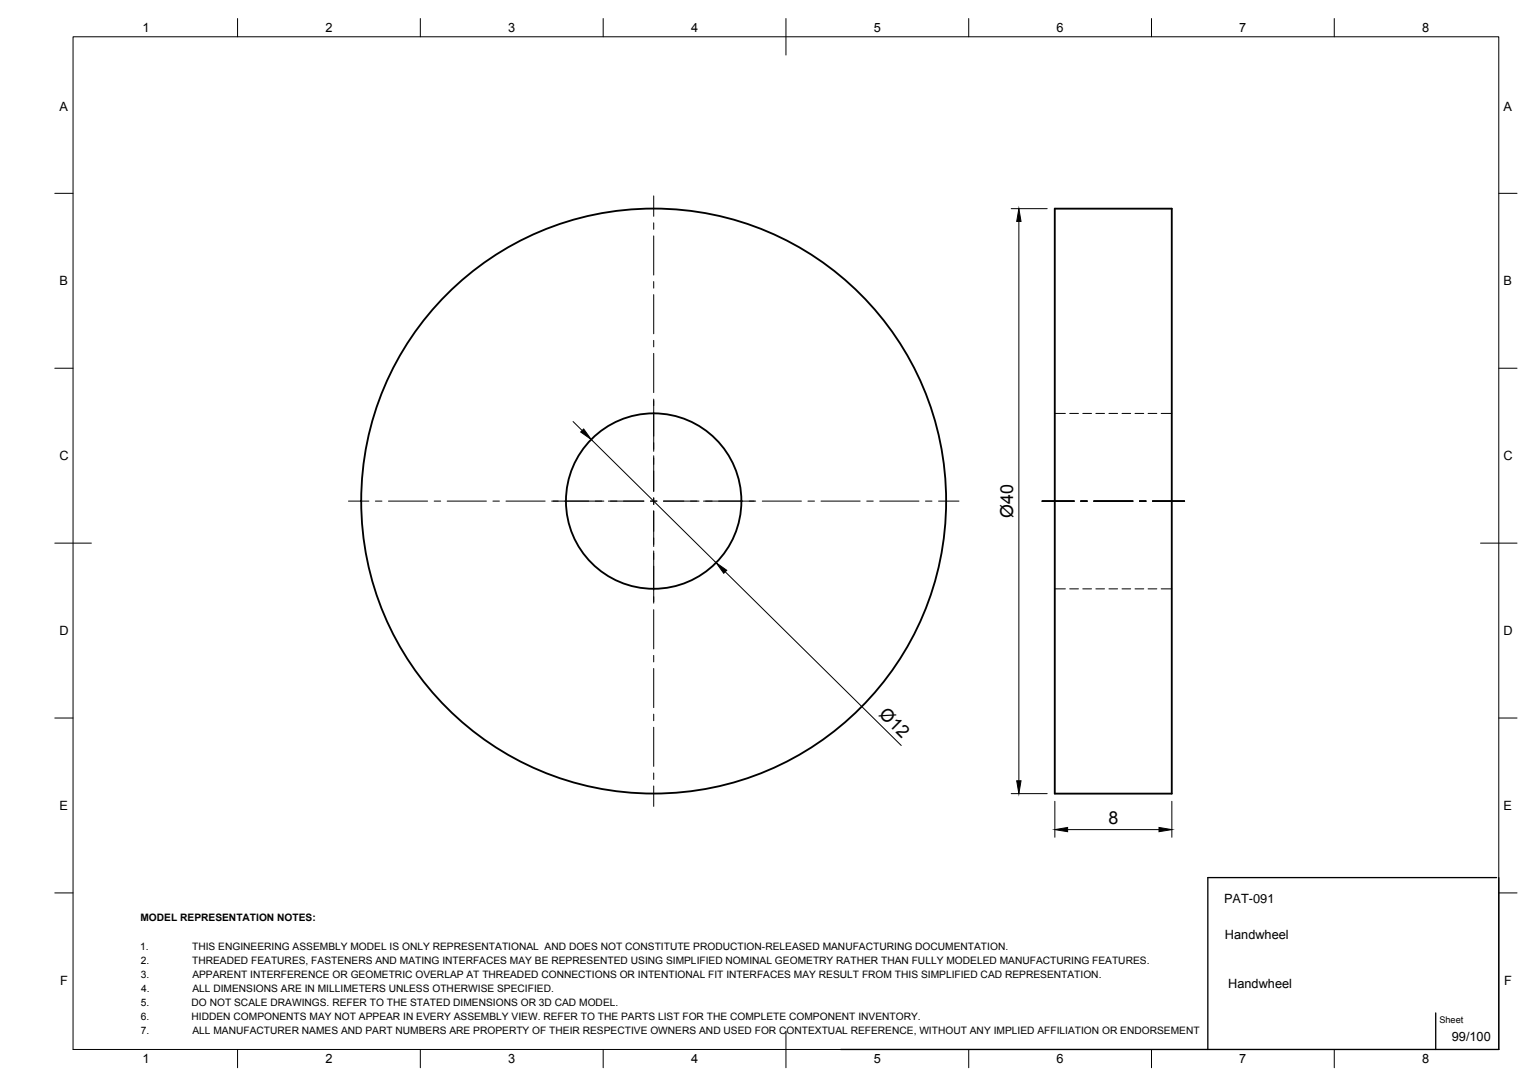
ISO-10303-21;
HEADER;
/* Generated by software containing ST-Developer
 * from STEP Tools, Inc. (www.steptools.com) 
 */

FILE_DESCRIPTION(
/* description */ ('PAT-091'),
/* implementation_level */ '2;1');

FILE_NAME(
/* name */ 'Handwheel.step',
/* time_stamp */ '2026-10-27T15:34:44-07:00',
/* author */ (''),
/* organization */ (''),
/* preprocessor_version */ 'ST-DEVELOPER v20.2',
/* originating_system */ 'Autodesk Translation Framework v15.17.0.0',
/* authorisation */ '');

FILE_SCHEMA (('AUTOMOTIVE_DESIGN { 1 0 10303 214 3 1 1 }'));
ENDSEC;

DATA;
#10=MECHANICAL_DESIGN_GEOMETRIC_PRESENTATION_REPRESENTATION('',(#1093),#25100);
#860=SHAPE_REPRESENTATION_RELATIONSHIP('SRR','None',#25629,#970);
#970=ADVANCED_BREP_SHAPE_REPRESENTATION('',(#1214),#25099);
#1093=STYLED_ITEM('',(#26184),#1214);
#1214=MANIFOLD_SOLID_BREP('Body1',#13373);
#1637=FACE_BOUND('',#4120,.T.);
#1638=FACE_BOUND('',#4122,.T.);
#1639=FACE_BOUND('',#4123,.T.);
#2060=PLANE('',#16445);
#2061=PLANE('',#16452);
#2062=PLANE('',#16453);
#2875=FACE_OUTER_BOUND('',#4115,.T.);
#2876=FACE_OUTER_BOUND('',#4116,.T.);
#2877=FACE_OUTER_BOUND('',#4117,.T.);
#2878=FACE_OUTER_BOUND('',#4118,.T.);
#2879=FACE_OUTER_BOUND('',#4119,.T.);
#2880=FACE_OUTER_BOUND('',#4121,.T.);
#4115=EDGE_LOOP('',(#12056,#12057,#12058,#12059));
#4116=EDGE_LOOP('',(#12060));
#4117=EDGE_LOOP('',(#12061,#12062,#12063,#12064));
#4118=EDGE_LOOP('',(#12065,#12066,#12067,#12068));
#4119=EDGE_LOOP('',(#12069));
#4120=EDGE_LOOP('',(#12070));
#4121=EDGE_LOOP('',(#12071));
#4122=EDGE_LOOP('',(#12072));
#4123=EDGE_LOOP('',(#12073));
#4861=LINE('',#24828,#5601);
#4862=LINE('',#24835,#5602);
#4863=LINE('',#24841,#5603);
#5601=VECTOR('',#20923,0.4);
#5602=VECTOR('',#20932,0.6);
#5603=VECTOR('',#20939,2.);
#6377=CIRCLE('',#16443,0.4);
#6378=CIRCLE('',#16444,0.4);
#6379=CIRCLE('',#16447,0.6);
#6380=CIRCLE('',#16448,0.6);
#6381=CIRCLE('',#16450,2.);
#6382=CIRCLE('',#16451,2.);
#7415=VERTEX_POINT('',#24825);
#7416=VERTEX_POINT('',#24827);
#7417=VERTEX_POINT('',#24832);
#7418=VERTEX_POINT('',#24834);
#7419=VERTEX_POINT('',#24838);
#7420=VERTEX_POINT('',#24840);
#8963=EDGE_CURVE('',#7415,#7415,#6377,.T.);
#8964=EDGE_CURVE('',#7415,#7416,#4861,.T.);
#8965=EDGE_CURVE('',#7416,#7416,#6378,.T.);
#8966=EDGE_CURVE('',#7417,#7417,#6379,.T.);
#8967=EDGE_CURVE('',#7417,#7418,#4862,.T.);
#8968=EDGE_CURVE('',#7418,#7418,#6380,.T.);
#8969=EDGE_CURVE('',#7419,#7419,#6381,.T.);
#8970=EDGE_CURVE('',#7419,#7420,#4863,.T.);
#8971=EDGE_CURVE('',#7420,#7420,#6382,.T.);
#12056=ORIENTED_EDGE('',*,*,#8963,.F.);
#12057=ORIENTED_EDGE('',*,*,#8964,.T.);
#12058=ORIENTED_EDGE('',*,*,#8965,.T.);
#12059=ORIENTED_EDGE('',*,*,#8964,.F.);
#12060=ORIENTED_EDGE('',*,*,#8965,.F.);
#12061=ORIENTED_EDGE('',*,*,#8966,.F.);
#12062=ORIENTED_EDGE('',*,*,#8967,.T.);
#12063=ORIENTED_EDGE('',*,*,#8968,.T.);
#12064=ORIENTED_EDGE('',*,*,#8967,.F.);
#12065=ORIENTED_EDGE('',*,*,#8969,.F.);
#12066=ORIENTED_EDGE('',*,*,#8970,.T.);
#12067=ORIENTED_EDGE('',*,*,#8971,.T.);
#12068=ORIENTED_EDGE('',*,*,#8970,.F.);
#12069=ORIENTED_EDGE('',*,*,#8969,.T.);
#12070=ORIENTED_EDGE('',*,*,#8966,.T.);
#12071=ORIENTED_EDGE('',*,*,#8971,.F.);
#12072=ORIENTED_EDGE('',*,*,#8963,.T.);
#12073=ORIENTED_EDGE('',*,*,#8968,.F.);
#12427=CYLINDRICAL_SURFACE('',#16442,0.4);
#12428=CYLINDRICAL_SURFACE('',#16446,0.6);
#12429=CYLINDRICAL_SURFACE('',#16449,2.);
#13242=ADVANCED_FACE('',(#2875),#12427,.T.);
#13243=ADVANCED_FACE('',(#2876),#2060,.F.);
#13244=ADVANCED_FACE('',(#2877),#12428,.F.);
#13245=ADVANCED_FACE('',(#2878),#12429,.T.);
#13246=ADVANCED_FACE('',(#2879,#1637),#2061,.T.);
#13247=ADVANCED_FACE('',(#2880,#1638,#1639),#2062,.F.);
#13373=CLOSED_SHELL('',(#13242,#13243,#13244,#13245,#13246,#13247));
#16441=AXIS2_PLACEMENT_3D('',#24823,#20917,#20918);
#16442=AXIS2_PLACEMENT_3D('',#24824,#20919,#20920);
#16443=AXIS2_PLACEMENT_3D('',#24826,#20921,#20922);
#16444=AXIS2_PLACEMENT_3D('',#24829,#20924,#20925);
#16445=AXIS2_PLACEMENT_3D('',#24830,#20926,#20927);
#16446=AXIS2_PLACEMENT_3D('',#24831,#20928,#20929);
#16447=AXIS2_PLACEMENT_3D('',#24833,#20930,#20931);
#16448=AXIS2_PLACEMENT_3D('',#24836,#20933,#20934);
#16449=AXIS2_PLACEMENT_3D('',#24837,#20935,#20936);
#16450=AXIS2_PLACEMENT_3D('',#24839,#20937,#20938);
#16451=AXIS2_PLACEMENT_3D('',#24842,#20940,#20941);
#16452=AXIS2_PLACEMENT_3D('',#24843,#20942,#20943);
#16453=AXIS2_PLACEMENT_3D('',#24844,#20944,#20945);
#20917=DIRECTION('axis',(0.,0.,1.));
#20918=DIRECTION('refdir',(1.,0.,0.));
#20919=DIRECTION('center_axis',(1.,0.,0.));
#20920=DIRECTION('ref_axis',(0.,0.,-1.));
#20921=DIRECTION('center_axis',(1.,0.,0.));
#20922=DIRECTION('ref_axis',(0.,0.,-1.));
#20923=DIRECTION('',(-1.,0.,0.));
#20924=DIRECTION('center_axis',(1.,0.,0.));
#20925=DIRECTION('ref_axis',(0.,0.,-1.));
#20926=DIRECTION('center_axis',(1.,0.,0.));
#20927=DIRECTION('ref_axis',(0.,0.,-1.));
#20928=DIRECTION('center_axis',(1.,0.,0.));
#20929=DIRECTION('ref_axis',(0.,0.,-1.));
#20930=DIRECTION('center_axis',(-1.,0.,0.));
#20931=DIRECTION('ref_axis',(0.,0.,-1.));
#20932=DIRECTION('',(-1.,0.,0.));
#20933=DIRECTION('center_axis',(-1.,0.,0.));
#20934=DIRECTION('ref_axis',(0.,0.,-1.));
#20935=DIRECTION('center_axis',(1.,0.,0.));
#20936=DIRECTION('ref_axis',(0.,0.,-1.));
#20937=DIRECTION('center_axis',(1.,0.,0.));
#20938=DIRECTION('ref_axis',(0.,0.,-1.));
#20939=DIRECTION('',(-1.,0.,0.));
#20940=DIRECTION('center_axis',(1.,0.,0.));
#20941=DIRECTION('ref_axis',(0.,0.,-1.));
#20942=DIRECTION('center_axis',(1.,0.,0.));
#20943=DIRECTION('ref_axis',(0.,0.,-1.));
#20944=DIRECTION('center_axis',(1.,0.,0.));
#20945=DIRECTION('ref_axis',(0.,0.,-1.));
#24823=CARTESIAN_POINT('',(0.,0.,0.));
#24824=CARTESIAN_POINT('Origin',(-5.5,0.,7.5));
#24825=CARTESIAN_POINT('',(-3.5,-4.89858719658942E-17,7.9));
#24826=CARTESIAN_POINT('Origin',(-3.5,0.,7.5));
#24827=CARTESIAN_POINT('',(-5.5,-4.89858719658942E-17,7.9));
#24828=CARTESIAN_POINT('',(-5.5,-4.89858719658942E-17,7.9));
#24829=CARTESIAN_POINT('Origin',(-5.5,0.,7.5));
#24830=CARTESIAN_POINT('Origin',(-5.5,0.,7.5));
#24831=CARTESIAN_POINT('Origin',(-3.5,0.,6.));
#24832=CARTESIAN_POINT('',(-2.7,-7.34788079488412E-17,6.6));
#24833=CARTESIAN_POINT('Origin',(-2.7,0.,6.));
#24834=CARTESIAN_POINT('',(-3.5,-7.34788079488412E-17,6.6));
#24835=CARTESIAN_POINT('',(-3.5,-7.34788079488412E-17,6.6));
#24836=CARTESIAN_POINT('Origin',(-3.5,0.,6.));
#24837=CARTESIAN_POINT('Origin',(-3.5,0.,6.));
#24838=CARTESIAN_POINT('',(-2.7,-2.44929359829471E-16,8.));
#24839=CARTESIAN_POINT('Origin',(-2.7,0.,6.));
#24840=CARTESIAN_POINT('',(-3.5,-2.44929359829471E-16,8.));
#24841=CARTESIAN_POINT('',(-3.5,-2.44929359829471E-16,8.));
#24842=CARTESIAN_POINT('Origin',(-3.5,0.,6.));
#24843=CARTESIAN_POINT('Origin',(-2.7,0.,6.));
#24844=CARTESIAN_POINT('Origin',(-3.5,0.,6.));
#24978=UNCERTAINTY_MEASURE_WITH_UNIT(LENGTH_MEASURE(0.001),#25101,
'DISTANCE_ACCURACY_VALUE',
'Maximum model space distance between geometric entities at asserted c
onnectivities');
#24979=UNCERTAINTY_MEASURE_WITH_UNIT(LENGTH_MEASURE(0.001),#25101,
'DISTANCE_ACCURACY_VALUE',
'Maximum model space distance between geometric entities at asserted c
onnectivities');
#25099=(
GEOMETRIC_REPRESENTATION_CONTEXT(3)
GLOBAL_UNCERTAINTY_ASSIGNED_CONTEXT((#24978))
GLOBAL_UNIT_ASSIGNED_CONTEXT((#25101,#25103,#25104))
REPRESENTATION_CONTEXT('','3D')
);
#25100=(
GEOMETRIC_REPRESENTATION_CONTEXT(3)
GLOBAL_UNCERTAINTY_ASSIGNED_CONTEXT((#24979))
GLOBAL_UNIT_ASSIGNED_CONTEXT((#25101,#25103,#25104))
REPRESENTATION_CONTEXT('','3D')
);
#25101=(
LENGTH_UNIT()
NAMED_UNIT(*)
SI_UNIT(.CENTI.,.METRE.)
);
#25103=(
NAMED_UNIT(*)
PLANE_ANGLE_UNIT()
SI_UNIT($,.RADIAN.)
);
#25104=(
NAMED_UNIT(*)
SI_UNIT($,.STERADIAN.)
SOLID_ANGLE_UNIT()
);
#25224=SHAPE_DEFINITION_REPRESENTATION(#25496,#25629);
#25496=PRODUCT_DEFINITION_SHAPE('',$,#25750);
#25629=SHAPE_REPRESENTATION('',(#16441),#25099);
#25630=PRODUCT_DEFINITION_CONTEXT('part definition',#25992,'design');
#25750=PRODUCT_DEFINITION('Handwheel','Handwheel',#25870,#25630);
#25870=PRODUCT_DEFINITION_FORMATION('',$,#26113);
#25992=APPLICATION_CONTEXT(
'Core Data for Automotive Mechanical Design Process');
#25993=PRODUCT_CONTEXT('part definition',#25992,'mechanical');
#26113=PRODUCT('Handwheel','Handwheel','Handwheel',(#25993));
#26178=COLOUR_RGB('Sky Blue',0.24,0.69,0.87);
#26179=FILL_AREA_STYLE_COLOUR('',#26178);
#26180=FILL_AREA_STYLE('',(#26179));
#26181=SURFACE_STYLE_FILL_AREA(#26180);
#26182=SURFACE_SIDE_STYLE('',(#26181));
#26183=SURFACE_STYLE_USAGE(.BOTH.,#26182);
#26184=PRESENTATION_STYLE_ASSIGNMENT((#26183));
ENDSEC;
END-ISO-10303-21;
